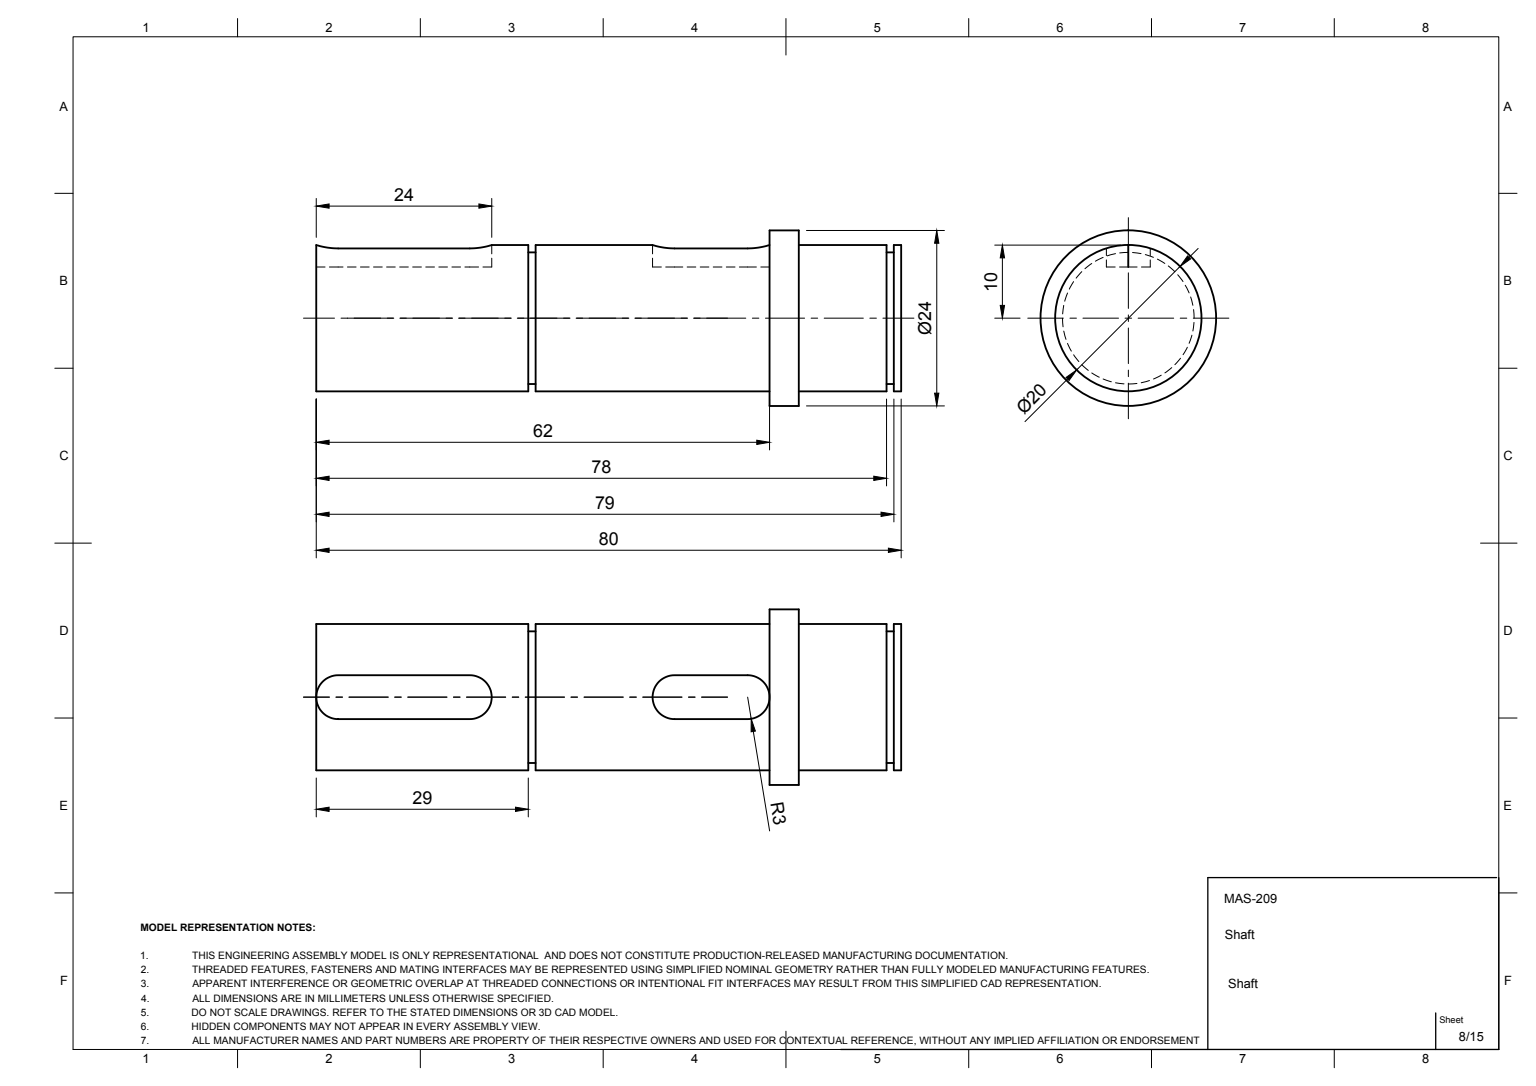
ISO-10303-21;
HEADER;
/* Generated by software containing ST-Developer
 * from STEP Tools, Inc. (www.steptools.com) 
 */

FILE_DESCRIPTION(
/* description */ ('Independent bearing-supported roller-ramp one-way clutch. Six logarit
hmic ramps with plain solid rollers, sprung guided plungers, native Co
il variants, removable shared keepers, rounded parallel key, shaft wit
h complete retaining lips, bronze journal/thrust support and bolted co
vers. Native rotor, roller planar/spin and plunger joints permit manua
l geometric engaged/released inspection. Automatic frictional torque s
witching/contact dynamics are not simulated; no capacity, hardness, fi
t, lubrication, speed, force or life rating. External input driver/cou
pling/anchors outside assembly.'),
/* implementation_level */ '2;1');

FILE_NAME(
/* name */ 'Shaft.step',
/* time_stamp */ '2026-11-08T07:04:38-08:00',
/* author */ (''),
/* organization */ (''),
/* preprocessor_version */ 'ST-DEVELOPER v20.2',
/* originating_system */ 'Autodesk Translation Framework v15.17.0.0',
/* authorisation */ '');

FILE_SCHEMA (('AUTOMOTIVE_DESIGN { 1 0 10303 214 3 1 1 }'));
ENDSEC;

DATA;
#10=MECHANICAL_DESIGN_GEOMETRIC_PRESENTATION_REPRESENTATION('',(#302),#99526);
#270=SHAPE_REPRESENTATION_RELATIONSHIP('SRR','None',#99627,#286);
#286=ADVANCED_BREP_SHAPE_REPRESENTATION('',(#318),#99512);
#302=STYLED_ITEM('',(#99716),#318);
#318=MANIFOLD_SOLID_BREP('Body1',#18272);
#388=FACE_BOUND('',#2557,.T.);
#389=FACE_BOUND('',#2559,.T.);
#390=FACE_BOUND('',#2562,.T.);
#391=FACE_BOUND('',#2564,.T.);
#392=FACE_BOUND('',#2567,.T.);
#393=FACE_BOUND('',#2569,.T.);
#547=PLANE('',#19435);
#548=PLANE('',#19438);
#549=PLANE('',#19439);
#550=PLANE('',#19446);
#551=PLANE('',#19449);
#552=PLANE('',#19450);
#553=PLANE('',#19458);
#554=PLANE('',#19459);
#555=PLANE('',#19463);
#556=PLANE('',#19465);
#557=PLANE('',#19469);
#558=PLANE('',#19471);
#559=PLANE('',#19476);
#560=PLANE('',#19477);
#1489=FACE_OUTER_BOUND('',#2542,.T.);
#1490=FACE_OUTER_BOUND('',#2543,.T.);
#1491=FACE_OUTER_BOUND('',#2544,.T.);
#1492=FACE_OUTER_BOUND('',#2545,.T.);
#1493=FACE_OUTER_BOUND('',#2546,.T.);
#1494=FACE_OUTER_BOUND('',#2547,.T.);
#1495=FACE_OUTER_BOUND('',#2548,.T.);
#1496=FACE_OUTER_BOUND('',#2549,.T.);
#1497=FACE_OUTER_BOUND('',#2550,.T.);
#1498=FACE_OUTER_BOUND('',#2551,.T.);
#1499=FACE_OUTER_BOUND('',#2552,.T.);
#1500=FACE_OUTER_BOUND('',#2553,.T.);
#1501=FACE_OUTER_BOUND('',#2554,.T.);
#1502=FACE_OUTER_BOUND('',#2555,.T.);
#1503=FACE_OUTER_BOUND('',#2556,.T.);
#1504=FACE_OUTER_BOUND('',#2558,.T.);
#1505=FACE_OUTER_BOUND('',#2560,.T.);
#1506=FACE_OUTER_BOUND('',#2561,.T.);
#1507=FACE_OUTER_BOUND('',#2563,.T.);
#1508=FACE_OUTER_BOUND('',#2565,.T.);
#1509=FACE_OUTER_BOUND('',#2566,.T.);
#1510=FACE_OUTER_BOUND('',#2568,.T.);
#1511=FACE_OUTER_BOUND('',#2570,.T.);
#1512=FACE_OUTER_BOUND('',#2571,.T.);
#1513=FACE_OUTER_BOUND('',#2572,.T.);
#1514=FACE_OUTER_BOUND('',#2573,.T.);
#2542=EDGE_LOOP('',(#15718,#15719,#15720,#15721));
#2543=EDGE_LOOP('',(#15722,#15723,#15724,#15725));
#2544=EDGE_LOOP('',(#15726,#15727,#15728,#15729));
#2545=EDGE_LOOP('',(#15730,#15731,#15732,#15733));
#2546=EDGE_LOOP('',(#15734,#15735,#15736,#15737));
#2547=EDGE_LOOP('',(#15738,#15739,#15740,#15741,#15742));
#2548=EDGE_LOOP('',(#15743,#15744,#15745,#15746,#15747,#15748,#15749,#15750,
#15751,#15752));
#2549=EDGE_LOOP('',(#15753,#15754,#15755,#15756));
#2550=EDGE_LOOP('',(#15757,#15758,#15759,#15760));
#2551=EDGE_LOOP('',(#15761,#15762,#15763,#15764,#15765));
#2552=EDGE_LOOP('',(#15766,#15767,#15768,#15769));
#2553=EDGE_LOOP('',(#15770,#15771,#15772,#15773));
#2554=EDGE_LOOP('',(#15774,#15775,#15776,#15777,#15778,#15779,#15780,#15781,
#15782,#15783));
#2555=EDGE_LOOP('',(#15784,#15785,#15786,#15787));
#2556=EDGE_LOOP('',(#15788));
#2557=EDGE_LOOP('',(#15789));
#2558=EDGE_LOOP('',(#15790));
#2559=EDGE_LOOP('',(#15791));
#2560=EDGE_LOOP('',(#15792,#15793,#15794,#15795));
#2561=EDGE_LOOP('',(#15796));
#2562=EDGE_LOOP('',(#15797));
#2563=EDGE_LOOP('',(#15798));
#2564=EDGE_LOOP('',(#15799));
#2565=EDGE_LOOP('',(#15800,#15801,#15802,#15803));
#2566=EDGE_LOOP('',(#15804));
#2567=EDGE_LOOP('',(#15805,#15806));
#2568=EDGE_LOOP('',(#15807));
#2569=EDGE_LOOP('',(#15808));
#2570=EDGE_LOOP('',(#15809,#15810,#15811,#15812));
#2571=EDGE_LOOP('',(#15813,#15814,#15815,#15816));
#2572=EDGE_LOOP('',(#15817,#15818,#15819,#15820));
#2573=EDGE_LOOP('',(#15821));
#2995=CIRCLE('',#19432,3.);
#2996=CIRCLE('',#19434,3.);
#2997=CIRCLE('',#19437,3.);
#2998=CIRCLE('',#19441,10.);
#2999=CIRCLE('',#19442,10.);
#3000=CIRCLE('',#19443,10.);
#3001=CIRCLE('',#19445,3.);
#3002=CIRCLE('',#19448,3.);
#3003=CIRCLE('',#19452,10.);
#3004=CIRCLE('',#19453,10.);
#3005=CIRCLE('',#19454,10.);
#3006=CIRCLE('',#19456,9.);
#3007=CIRCLE('',#19457,9.);
#3008=CIRCLE('',#19461,9.);
#3009=CIRCLE('',#19462,9.);
#3010=CIRCLE('',#19464,10.);
#3011=CIRCLE('',#19466,10.);
#3012=CIRCLE('',#19468,10.);
#3013=CIRCLE('',#19470,12.);
#3014=CIRCLE('',#19472,12.);
#3015=CIRCLE('',#19475,10.);
#4509=B_SPLINE_CURVE_WITH_KNOTS('',3,(#94457,#94458,#94459,#94460,#94461,
#94462,#94463,#94464,#94465,#94466),.UNSPECIFIED.,.F.,.F.,(4,2,2,2,4),(-0.455064911568751,
-0.34131563198115,-0.227566352393549,-0.113783176196775,0.),
 .UNSPECIFIED.);
#4510=B_SPLINE_CURVE_WITH_KNOTS('',3,(#94469,#94470,#94471,#94472,#94473,
#94474,#94475,#94476,#94477,#94478),.UNSPECIFIED.,.F.,.F.,(4,2,2,2,4),(-0.910129823137502,
-0.796346646940727,-0.682563470743952,-0.568814191156351,-0.455064911568751),
 .UNSPECIFIED.);
#4511=B_SPLINE_CURVE_WITH_KNOTS('',3,(#94491,#94492,#94493,#94494,#94495,
#94496,#94497,#94498,#94499,#94500,#94501,#94502,#94503,#94504,#94505,#94506,
#94507,#94508),.UNSPECIFIED.,.F.,.F.,(4,2,2,2,2,2,2,2,4),(0.,0.113783176196775,
0.227566352393549,0.34131563198115,0.455064911568751,0.568814191156351,
0.682563470743952,0.796346646940727,0.910129823137502),.UNSPECIFIED.);
#4512=B_SPLINE_CURVE_WITH_KNOTS('',3,(#94526,#94527,#94528,#94529,#94530,
#94531,#94532,#94533,#94534,#94535,#94536,#94537,#94538,#94539,#94540,#94541,
#94542,#94543),.UNSPECIFIED.,.F.,.F.,(4,2,2,2,2,2,2,2,4),(-0.910129823137503,
-0.796346646940728,-0.682563470743953,-0.568814191156352,-0.455064911568751,
-0.341315631981151,-0.22756635239355,-0.113783176196775,0.),
 .UNSPECIFIED.);
#4513=B_SPLINE_CURVE_WITH_KNOTS('',3,(#94558,#94559,#94560,#94561,#94562,
#94563,#94564,#94565,#94566,#94567),.UNSPECIFIED.,.F.,.F.,(4,2,2,2,4),(0.455064911568751,
0.568814191156352,0.682563470743953,0.796346646940727,0.910129823137502),
 .UNSPECIFIED.);
#4514=B_SPLINE_CURVE_WITH_KNOTS('',3,(#94568,#94569,#94570,#94571,#94572,
#94573,#94574,#94575,#94576,#94577),.UNSPECIFIED.,.F.,.F.,(4,2,2,2,4),(0.,
0.113783176196775,0.22756635239355,0.341315631981151,0.455064911568751),
 .UNSPECIFIED.);
#5366=LINE('',#94452,#6270);
#5367=LINE('',#94456,#6271);
#5368=LINE('',#94480,#6272);
#5369=LINE('',#94482,#6273);
#5370=LINE('',#94485,#6274);
#5371=LINE('',#94487,#6275);
#5372=LINE('',#94488,#6276);
#5373=LINE('',#94511,#6277);
#5374=LINE('',#94513,#6278);
#5375=LINE('',#94514,#6279);
#5376=LINE('',#94521,#6280);
#5377=LINE('',#94545,#6281);
#5378=LINE('',#94548,#6282);
#5379=LINE('',#94551,#6283);
#5380=LINE('',#94553,#6284);
#5381=LINE('',#94554,#6285);
#5382=LINE('',#94580,#6286);
#5383=LINE('',#94582,#6287);
#5384=LINE('',#94583,#6288);
#5385=LINE('',#94589,#6289);
#5386=LINE('',#94596,#6290);
#5387=LINE('',#94604,#6291);
#5388=LINE('',#94615,#6292);
#5389=LINE('',#94623,#6293);
#5390=LINE('',#94626,#6294);
#6270=VECTOR('',#22473,10.);
#6271=VECTOR('',#22476,10.);
#6272=VECTOR('',#22479,10.);
#6273=VECTOR('',#22482,10.);
#6274=VECTOR('',#22485,10.);
#6275=VECTOR('',#22486,10.);
#6276=VECTOR('',#22487,10.);
#6277=VECTOR('',#22492,10.);
#6278=VECTOR('',#22495,10.);
#6279=VECTOR('',#22496,10.);
#6280=VECTOR('',#22505,10.);
#6281=VECTOR('',#22510,10.);
#6282=VECTOR('',#22513,10.);
#6283=VECTOR('',#22516,10.);
#6284=VECTOR('',#22517,10.);
#6285=VECTOR('',#22518,10.);
#6286=VECTOR('',#22523,10.);
#6287=VECTOR('',#22526,10.);
#6288=VECTOR('',#22527,10.);
#6289=VECTOR('',#22534,10.);
#6290=VECTOR('',#22543,9.);
#6291=VECTOR('',#22554,9.);
#6292=VECTOR('',#22569,10.);
#6293=VECTOR('',#22580,12.);
#6294=VECTOR('',#22583,10.);
#7994=VERTEX_POINT('',#94450);
#7995=VERTEX_POINT('',#94451);
#7996=VERTEX_POINT('',#94453);
#7997=VERTEX_POINT('',#94455);
#7998=VERTEX_POINT('',#94468);
#7999=VERTEX_POINT('',#94479);
#8000=VERTEX_POINT('',#94484);
#8001=VERTEX_POINT('',#94486);
#8002=VERTEX_POINT('',#94490);
#8003=VERTEX_POINT('',#94509);
#8004=VERTEX_POINT('',#94517);
#8005=VERTEX_POINT('',#94520);
#8006=VERTEX_POINT('',#94524);
#8007=VERTEX_POINT('',#94525);
#8008=VERTEX_POINT('',#94544);
#8009=VERTEX_POINT('',#94546);
#8010=VERTEX_POINT('',#94550);
#8011=VERTEX_POINT('',#94552);
#8012=VERTEX_POINT('',#94556);
#8013=VERTEX_POINT('',#94557);
#8014=VERTEX_POINT('',#94578);
#8015=VERTEX_POINT('',#94586);
#8016=VERTEX_POINT('',#94588);
#8017=VERTEX_POINT('',#94593);
#8018=VERTEX_POINT('',#94595);
#8019=VERTEX_POINT('',#94601);
#8020=VERTEX_POINT('',#94603);
#8021=VERTEX_POINT('',#94607);
#8022=VERTEX_POINT('',#94610);
#8023=VERTEX_POINT('',#94613);
#8024=VERTEX_POINT('',#94617);
#8025=VERTEX_POINT('',#94620);
#8026=VERTEX_POINT('',#94625);
#10611=EDGE_CURVE('',#7994,#7995,#5366,.T.);
#10612=EDGE_CURVE('',#7996,#7994,#2995,.T.);
#10613=EDGE_CURVE('',#7996,#7997,#5367,.T.);
#10614=EDGE_CURVE('',#7995,#7997,#4509,.T.);
#10615=EDGE_CURVE('',#7998,#7995,#4510,.T.);
#10616=EDGE_CURVE('',#7999,#7998,#5368,.T.);
#10617=EDGE_CURVE('',#7994,#7999,#2996,.T.);
#10618=EDGE_CURVE('',#7994,#7995,#5369,.T.);
#10619=EDGE_CURVE('',#7997,#8000,#5370,.T.);
#10620=EDGE_CURVE('',#7996,#8001,#5371,.T.);
#10621=EDGE_CURVE('',#8001,#8000,#5372,.T.);
#10622=EDGE_CURVE('',#8000,#8002,#4511,.T.);
#10623=EDGE_CURVE('',#8003,#8001,#2997,.T.);
#10624=EDGE_CURVE('',#8003,#8002,#5373,.T.);
#10625=EDGE_CURVE('',#8002,#7998,#5374,.T.);
#10626=EDGE_CURVE('',#8003,#7999,#5375,.T.);
#10627=EDGE_CURVE('',#7995,#8004,#2998,.T.);
#10628=EDGE_CURVE('',#8004,#7995,#2999,.T.);
#10629=EDGE_CURVE('',#8004,#8005,#5376,.T.);
#10630=EDGE_CURVE('',#8005,#8005,#3000,.T.);
#10631=EDGE_CURVE('',#8006,#8007,#4512,.T.);
#10632=EDGE_CURVE('',#8008,#8006,#5377,.T.);
#10633=EDGE_CURVE('',#8009,#8008,#3001,.T.);
#10634=EDGE_CURVE('',#8009,#8007,#5378,.T.);
#10635=EDGE_CURVE('',#8007,#8010,#5379,.T.);
#10636=EDGE_CURVE('',#8009,#8011,#5380,.T.);
#10637=EDGE_CURVE('',#8011,#8010,#5381,.T.);
#10638=EDGE_CURVE('',#8012,#8013,#4513,.T.);
#10639=EDGE_CURVE('',#8010,#8012,#4514,.T.);
#10640=EDGE_CURVE('',#8014,#8011,#3002,.T.);
#10641=EDGE_CURVE('',#8014,#8013,#5382,.T.);
#10642=EDGE_CURVE('',#8013,#8006,#5383,.T.);
#10643=EDGE_CURVE('',#8014,#8008,#5384,.T.);
#10644=EDGE_CURVE('',#8015,#8015,#3003,.T.);
#10645=EDGE_CURVE('',#8015,#8016,#5385,.T.);
#10646=EDGE_CURVE('',#8016,#8012,#3004,.T.);
#10647=EDGE_CURVE('',#8012,#8016,#3005,.T.);
#10648=EDGE_CURVE('',#8017,#8017,#3006,.T.);
#10649=EDGE_CURVE('',#8017,#8018,#5386,.T.);
#10650=EDGE_CURVE('',#8018,#8018,#3007,.T.);
#10651=EDGE_CURVE('',#8019,#8019,#3008,.T.);
#10652=EDGE_CURVE('',#8019,#8020,#5387,.T.);
#10653=EDGE_CURVE('',#8020,#8020,#3009,.T.);
#10654=EDGE_CURVE('',#8021,#8021,#3010,.T.);
#10655=EDGE_CURVE('',#8022,#8022,#3011,.T.);
#10656=EDGE_CURVE('',#8023,#8023,#3012,.T.);
#10657=EDGE_CURVE('',#8023,#8022,#5388,.T.);
#10658=EDGE_CURVE('',#8024,#8024,#3013,.T.);
#10659=EDGE_CURVE('',#8025,#8025,#3014,.T.);
#10660=EDGE_CURVE('',#8024,#8025,#5389,.T.);
#10661=EDGE_CURVE('',#8021,#8026,#5390,.T.);
#10662=EDGE_CURVE('',#8026,#8026,#3015,.T.);
#15718=ORIENTED_EDGE('',*,*,#10611,.F.);
#15719=ORIENTED_EDGE('',*,*,#10612,.F.);
#15720=ORIENTED_EDGE('',*,*,#10613,.T.);
#15721=ORIENTED_EDGE('',*,*,#10614,.F.);
#15722=ORIENTED_EDGE('',*,*,#10615,.F.);
#15723=ORIENTED_EDGE('',*,*,#10616,.F.);
#15724=ORIENTED_EDGE('',*,*,#10617,.F.);
#15725=ORIENTED_EDGE('',*,*,#10618,.T.);
#15726=ORIENTED_EDGE('',*,*,#10619,.F.);
#15727=ORIENTED_EDGE('',*,*,#10613,.F.);
#15728=ORIENTED_EDGE('',*,*,#10620,.T.);
#15729=ORIENTED_EDGE('',*,*,#10621,.T.);
#15730=ORIENTED_EDGE('',*,*,#10622,.F.);
#15731=ORIENTED_EDGE('',*,*,#10621,.F.);
#15732=ORIENTED_EDGE('',*,*,#10623,.F.);
#15733=ORIENTED_EDGE('',*,*,#10624,.T.);
#15734=ORIENTED_EDGE('',*,*,#10625,.F.);
#15735=ORIENTED_EDGE('',*,*,#10624,.F.);
#15736=ORIENTED_EDGE('',*,*,#10626,.T.);
#15737=ORIENTED_EDGE('',*,*,#10616,.T.);
#15738=ORIENTED_EDGE('',*,*,#10612,.T.);
#15739=ORIENTED_EDGE('',*,*,#10617,.T.);
#15740=ORIENTED_EDGE('',*,*,#10626,.F.);
#15741=ORIENTED_EDGE('',*,*,#10623,.T.);
#15742=ORIENTED_EDGE('',*,*,#10620,.F.);
#15743=ORIENTED_EDGE('',*,*,#10627,.F.);
#15744=ORIENTED_EDGE('',*,*,#10614,.T.);
#15745=ORIENTED_EDGE('',*,*,#10619,.T.);
#15746=ORIENTED_EDGE('',*,*,#10622,.T.);
#15747=ORIENTED_EDGE('',*,*,#10625,.T.);
#15748=ORIENTED_EDGE('',*,*,#10615,.T.);
#15749=ORIENTED_EDGE('',*,*,#10628,.F.);
#15750=ORIENTED_EDGE('',*,*,#10629,.T.);
#15751=ORIENTED_EDGE('',*,*,#10630,.T.);
#15752=ORIENTED_EDGE('',*,*,#10629,.F.);
#15753=ORIENTED_EDGE('',*,*,#10631,.F.);
#15754=ORIENTED_EDGE('',*,*,#10632,.F.);
#15755=ORIENTED_EDGE('',*,*,#10633,.F.);
#15756=ORIENTED_EDGE('',*,*,#10634,.T.);
#15757=ORIENTED_EDGE('',*,*,#10635,.F.);
#15758=ORIENTED_EDGE('',*,*,#10634,.F.);
#15759=ORIENTED_EDGE('',*,*,#10636,.T.);
#15760=ORIENTED_EDGE('',*,*,#10637,.T.);
#15761=ORIENTED_EDGE('',*,*,#10638,.F.);
#15762=ORIENTED_EDGE('',*,*,#10639,.F.);
#15763=ORIENTED_EDGE('',*,*,#10637,.F.);
#15764=ORIENTED_EDGE('',*,*,#10640,.F.);
#15765=ORIENTED_EDGE('',*,*,#10641,.T.);
#15766=ORIENTED_EDGE('',*,*,#10642,.F.);
#15767=ORIENTED_EDGE('',*,*,#10641,.F.);
#15768=ORIENTED_EDGE('',*,*,#10643,.T.);
#15769=ORIENTED_EDGE('',*,*,#10632,.T.);
#15770=ORIENTED_EDGE('',*,*,#10633,.T.);
#15771=ORIENTED_EDGE('',*,*,#10643,.F.);
#15772=ORIENTED_EDGE('',*,*,#10640,.T.);
#15773=ORIENTED_EDGE('',*,*,#10636,.F.);
#15774=ORIENTED_EDGE('',*,*,#10644,.T.);
#15775=ORIENTED_EDGE('',*,*,#10645,.T.);
#15776=ORIENTED_EDGE('',*,*,#10646,.T.);
#15777=ORIENTED_EDGE('',*,*,#10638,.T.);
#15778=ORIENTED_EDGE('',*,*,#10642,.T.);
#15779=ORIENTED_EDGE('',*,*,#10631,.T.);
#15780=ORIENTED_EDGE('',*,*,#10635,.T.);
#15781=ORIENTED_EDGE('',*,*,#10639,.T.);
#15782=ORIENTED_EDGE('',*,*,#10647,.T.);
#15783=ORIENTED_EDGE('',*,*,#10645,.F.);
#15784=ORIENTED_EDGE('',*,*,#10648,.T.);
#15785=ORIENTED_EDGE('',*,*,#10649,.T.);
#15786=ORIENTED_EDGE('',*,*,#10650,.F.);
#15787=ORIENTED_EDGE('',*,*,#10649,.F.);
#15788=ORIENTED_EDGE('',*,*,#10644,.F.);
#15789=ORIENTED_EDGE('',*,*,#10648,.F.);
#15790=ORIENTED_EDGE('',*,*,#10630,.F.);
#15791=ORIENTED_EDGE('',*,*,#10650,.T.);
#15792=ORIENTED_EDGE('',*,*,#10651,.T.);
#15793=ORIENTED_EDGE('',*,*,#10652,.T.);
#15794=ORIENTED_EDGE('',*,*,#10653,.F.);
#15795=ORIENTED_EDGE('',*,*,#10652,.F.);
#15796=ORIENTED_EDGE('',*,*,#10654,.F.);
#15797=ORIENTED_EDGE('',*,*,#10651,.F.);
#15798=ORIENTED_EDGE('',*,*,#10655,.F.);
#15799=ORIENTED_EDGE('',*,*,#10653,.T.);
#15800=ORIENTED_EDGE('',*,*,#10656,.T.);
#15801=ORIENTED_EDGE('',*,*,#10657,.T.);
#15802=ORIENTED_EDGE('',*,*,#10655,.T.);
#15803=ORIENTED_EDGE('',*,*,#10657,.F.);
#15804=ORIENTED_EDGE('',*,*,#10658,.T.);
#15805=ORIENTED_EDGE('',*,*,#10647,.F.);
#15806=ORIENTED_EDGE('',*,*,#10646,.F.);
#15807=ORIENTED_EDGE('',*,*,#10659,.F.);
#15808=ORIENTED_EDGE('',*,*,#10656,.F.);
#15809=ORIENTED_EDGE('',*,*,#10658,.F.);
#15810=ORIENTED_EDGE('',*,*,#10660,.T.);
#15811=ORIENTED_EDGE('',*,*,#10659,.T.);
#15812=ORIENTED_EDGE('',*,*,#10660,.F.);
#15813=ORIENTED_EDGE('',*,*,#10654,.T.);
#15814=ORIENTED_EDGE('',*,*,#10661,.T.);
#15815=ORIENTED_EDGE('',*,*,#10662,.T.);
#15816=ORIENTED_EDGE('',*,*,#10661,.F.);
#15817=ORIENTED_EDGE('',*,*,#10627,.T.);
#15818=ORIENTED_EDGE('',*,*,#10628,.T.);
#15819=ORIENTED_EDGE('',*,*,#10618,.F.);
#15820=ORIENTED_EDGE('',*,*,#10611,.T.);
#15821=ORIENTED_EDGE('',*,*,#10662,.F.);
#17171=CYLINDRICAL_SURFACE('',#19431,3.);
#17172=CYLINDRICAL_SURFACE('',#19433,3.);
#17173=CYLINDRICAL_SURFACE('',#19436,3.);
#17174=CYLINDRICAL_SURFACE('',#19440,10.);
#17175=CYLINDRICAL_SURFACE('',#19444,3.);
#17176=CYLINDRICAL_SURFACE('',#19447,3.);
#17177=CYLINDRICAL_SURFACE('',#19451,10.);
#17178=CYLINDRICAL_SURFACE('',#19455,9.);
#17179=CYLINDRICAL_SURFACE('',#19460,9.);
#17180=CYLINDRICAL_SURFACE('',#19467,10.);
#17181=CYLINDRICAL_SURFACE('',#19473,12.);
#17182=CYLINDRICAL_SURFACE('',#19474,10.);
#18087=ADVANCED_FACE('',(#1489),#17171,.F.);
#18088=ADVANCED_FACE('',(#1490),#17172,.F.);
#18089=ADVANCED_FACE('',(#1491),#547,.F.);
#18090=ADVANCED_FACE('',(#1492),#17173,.F.);
#18091=ADVANCED_FACE('',(#1493),#548,.F.);
#18092=ADVANCED_FACE('',(#1494),#549,.T.);
#18093=ADVANCED_FACE('',(#1495),#17174,.T.);
#18094=ADVANCED_FACE('',(#1496),#17175,.F.);
#18095=ADVANCED_FACE('',(#1497),#550,.F.);
#18096=ADVANCED_FACE('',(#1498),#17176,.F.);
#18097=ADVANCED_FACE('',(#1499),#551,.F.);
#18098=ADVANCED_FACE('',(#1500),#552,.T.);
#18099=ADVANCED_FACE('',(#1501),#17177,.T.);
#18100=ADVANCED_FACE('',(#1502),#17178,.T.);
#18101=ADVANCED_FACE('',(#1503,#388),#553,.F.);
#18102=ADVANCED_FACE('',(#1504,#389),#554,.F.);
#18103=ADVANCED_FACE('',(#1505),#17179,.T.);
#18104=ADVANCED_FACE('',(#1506,#390),#555,.F.);
#18105=ADVANCED_FACE('',(#1507,#391),#556,.F.);
#18106=ADVANCED_FACE('',(#1508),#17180,.T.);
#18107=ADVANCED_FACE('',(#1509,#392),#557,.T.);
#18108=ADVANCED_FACE('',(#1510,#393),#558,.F.);
#18109=ADVANCED_FACE('',(#1511),#17181,.T.);
#18110=ADVANCED_FACE('',(#1512),#17182,.T.);
#18111=ADVANCED_FACE('',(#1513),#559,.T.);
#18112=ADVANCED_FACE('',(#1514),#560,.F.);
#18272=CLOSED_SHELL('',(#18087,#18088,#18089,#18090,#18091,#18092,#18093,
#18094,#18095,#18096,#18097,#18098,#18099,#18100,#18101,#18102,#18103,#18104,
#18105,#18106,#18107,#18108,#18109,#18110,#18111,#18112));
#19430=AXIS2_PLACEMENT_3D('',#94448,#22469,#22470);
#19431=AXIS2_PLACEMENT_3D('',#94449,#22471,#22472);
#19432=AXIS2_PLACEMENT_3D('',#94454,#22474,#22475);
#19433=AXIS2_PLACEMENT_3D('',#94467,#22477,#22478);
#19434=AXIS2_PLACEMENT_3D('',#94481,#22480,#22481);
#19435=AXIS2_PLACEMENT_3D('',#94483,#22483,#22484);
#19436=AXIS2_PLACEMENT_3D('',#94489,#22488,#22489);
#19437=AXIS2_PLACEMENT_3D('',#94510,#22490,#22491);
#19438=AXIS2_PLACEMENT_3D('',#94512,#22493,#22494);
#19439=AXIS2_PLACEMENT_3D('',#94515,#22497,#22498);
#19440=AXIS2_PLACEMENT_3D('',#94516,#22499,#22500);
#19441=AXIS2_PLACEMENT_3D('',#94518,#22501,#22502);
#19442=AXIS2_PLACEMENT_3D('',#94519,#22503,#22504);
#19443=AXIS2_PLACEMENT_3D('',#94522,#22506,#22507);
#19444=AXIS2_PLACEMENT_3D('',#94523,#22508,#22509);
#19445=AXIS2_PLACEMENT_3D('',#94547,#22511,#22512);
#19446=AXIS2_PLACEMENT_3D('',#94549,#22514,#22515);
#19447=AXIS2_PLACEMENT_3D('',#94555,#22519,#22520);
#19448=AXIS2_PLACEMENT_3D('',#94579,#22521,#22522);
#19449=AXIS2_PLACEMENT_3D('',#94581,#22524,#22525);
#19450=AXIS2_PLACEMENT_3D('',#94584,#22528,#22529);
#19451=AXIS2_PLACEMENT_3D('',#94585,#22530,#22531);
#19452=AXIS2_PLACEMENT_3D('',#94587,#22532,#22533);
#19453=AXIS2_PLACEMENT_3D('',#94590,#22535,#22536);
#19454=AXIS2_PLACEMENT_3D('',#94591,#22537,#22538);
#19455=AXIS2_PLACEMENT_3D('',#94592,#22539,#22540);
#19456=AXIS2_PLACEMENT_3D('',#94594,#22541,#22542);
#19457=AXIS2_PLACEMENT_3D('',#94597,#22544,#22545);
#19458=AXIS2_PLACEMENT_3D('',#94598,#22546,#22547);
#19459=AXIS2_PLACEMENT_3D('',#94599,#22548,#22549);
#19460=AXIS2_PLACEMENT_3D('',#94600,#22550,#22551);
#19461=AXIS2_PLACEMENT_3D('',#94602,#22552,#22553);
#19462=AXIS2_PLACEMENT_3D('',#94605,#22555,#22556);
#19463=AXIS2_PLACEMENT_3D('',#94606,#22557,#22558);
#19464=AXIS2_PLACEMENT_3D('',#94608,#22559,#22560);
#19465=AXIS2_PLACEMENT_3D('',#94609,#22561,#22562);
#19466=AXIS2_PLACEMENT_3D('',#94611,#22563,#22564);
#19467=AXIS2_PLACEMENT_3D('',#94612,#22565,#22566);
#19468=AXIS2_PLACEMENT_3D('',#94614,#22567,#22568);
#19469=AXIS2_PLACEMENT_3D('',#94616,#22570,#22571);
#19470=AXIS2_PLACEMENT_3D('',#94618,#22572,#22573);
#19471=AXIS2_PLACEMENT_3D('',#94619,#22574,#22575);
#19472=AXIS2_PLACEMENT_3D('',#94621,#22576,#22577);
#19473=AXIS2_PLACEMENT_3D('',#94622,#22578,#22579);
#19474=AXIS2_PLACEMENT_3D('',#94624,#22581,#22582);
#19475=AXIS2_PLACEMENT_3D('',#94627,#22584,#22585);
#19476=AXIS2_PLACEMENT_3D('',#94628,#22586,#22587);
#19477=AXIS2_PLACEMENT_3D('',#94629,#22588,#22589);
#22469=DIRECTION('axis',(0.,0.,1.));
#22470=DIRECTION('refdir',(1.,0.,0.));
#22471=DIRECTION('center_axis',(1.,0.,0.));
#22472=DIRECTION('ref_axis',(0.,1.,-2.96059473233375E-15));
#22473=DIRECTION('',(1.,0.,0.));
#22474=DIRECTION('center_axis',(1.,0.,0.));
#22475=DIRECTION('ref_axis',(0.,1.,-2.96059473233375E-15));
#22476=DIRECTION('',(1.,0.,0.));
#22477=DIRECTION('center_axis',(1.,0.,0.));
#22478=DIRECTION('ref_axis',(0.,1.,-2.96059473233375E-15));
#22479=DIRECTION('',(1.,0.,0.));
#22480=DIRECTION('center_axis',(1.,0.,0.));
#22481=DIRECTION('ref_axis',(0.,1.,-2.96059473233375E-15));
#22482=DIRECTION('',(1.,0.,0.));
#22483=DIRECTION('center_axis',(0.,1.,0.));
#22484=DIRECTION('ref_axis',(0.,0.,1.));
#22485=DIRECTION('',(0.,0.,-1.));
#22486=DIRECTION('',(0.,0.,-1.));
#22487=DIRECTION('',(1.,0.,0.));
#22488=DIRECTION('center_axis',(1.,0.,0.));
#22489=DIRECTION('ref_axis',(0.,-1.,-2.96059473233375E-15));
#22490=DIRECTION('center_axis',(1.,0.,0.));
#22491=DIRECTION('ref_axis',(0.,-1.,-2.96059473233375E-15));
#22492=DIRECTION('',(1.,0.,0.));
#22493=DIRECTION('center_axis',(0.,-1.,0.));
#22494=DIRECTION('ref_axis',(0.,0.,-1.));
#22495=DIRECTION('',(0.,0.,1.));
#22496=DIRECTION('',(0.,0.,1.));
#22497=DIRECTION('center_axis',(1.,0.,0.));
#22498=DIRECTION('ref_axis',(0.,0.,-1.));
#22499=DIRECTION('center_axis',(0.,0.,1.));
#22500=DIRECTION('ref_axis',(1.,0.,0.));
#22501=DIRECTION('center_axis',(0.,0.,1.));
#22502=DIRECTION('ref_axis',(1.,0.,0.));
#22503=DIRECTION('center_axis',(0.,0.,1.));
#22504=DIRECTION('ref_axis',(1.,0.,0.));
#22505=DIRECTION('',(0.,0.,-1.));
#22506=DIRECTION('center_axis',(0.,0.,1.));
#22507=DIRECTION('ref_axis',(1.,0.,0.));
#22508=DIRECTION('center_axis',(1.,0.,0.));
#22509=DIRECTION('ref_axis',(0.,1.,0.));
#22510=DIRECTION('',(1.,0.,0.));
#22511=DIRECTION('center_axis',(1.,0.,0.));
#22512=DIRECTION('ref_axis',(0.,1.,0.));
#22513=DIRECTION('',(1.,0.,0.));
#22514=DIRECTION('center_axis',(0.,1.,0.));
#22515=DIRECTION('ref_axis',(0.,0.,1.));
#22516=DIRECTION('',(0.,0.,-1.));
#22517=DIRECTION('',(0.,0.,-1.));
#22518=DIRECTION('',(1.,0.,0.));
#22519=DIRECTION('center_axis',(1.,0.,0.));
#22520=DIRECTION('ref_axis',(0.,-1.,0.));
#22521=DIRECTION('center_axis',(1.,0.,0.));
#22522=DIRECTION('ref_axis',(0.,-1.,0.));
#22523=DIRECTION('',(1.,0.,0.));
#22524=DIRECTION('center_axis',(0.,-1.,0.));
#22525=DIRECTION('ref_axis',(0.,0.,-1.));
#22526=DIRECTION('',(0.,0.,1.));
#22527=DIRECTION('',(0.,0.,1.));
#22528=DIRECTION('center_axis',(1.,0.,0.));
#22529=DIRECTION('ref_axis',(0.,0.,-1.));
#22530=DIRECTION('center_axis',(0.,0.,1.));
#22531=DIRECTION('ref_axis',(1.,0.,0.));
#22532=DIRECTION('center_axis',(0.,0.,-1.));
#22533=DIRECTION('ref_axis',(1.,0.,0.));
#22534=DIRECTION('',(0.,0.,-1.));
#22535=DIRECTION('center_axis',(0.,0.,1.));
#22536=DIRECTION('ref_axis',(1.,0.,0.));
#22537=DIRECTION('center_axis',(0.,0.,1.));
#22538=DIRECTION('ref_axis',(1.,0.,0.));
#22539=DIRECTION('center_axis',(0.,0.,1.));
#22540=DIRECTION('ref_axis',(1.,0.,0.));
#22541=DIRECTION('center_axis',(0.,0.,1.));
#22542=DIRECTION('ref_axis',(1.,0.,0.));
#22543=DIRECTION('',(0.,0.,1.));
#22544=DIRECTION('center_axis',(0.,0.,1.));
#22545=DIRECTION('ref_axis',(1.,0.,0.));
#22546=DIRECTION('center_axis',(0.,0.,-1.));
#22547=DIRECTION('ref_axis',(-1.,0.,0.));
#22548=DIRECTION('center_axis',(0.,0.,1.));
#22549=DIRECTION('ref_axis',(1.,0.,0.));
#22550=DIRECTION('center_axis',(0.,0.,1.));
#22551=DIRECTION('ref_axis',(1.,0.,0.));
#22552=DIRECTION('center_axis',(0.,0.,1.));
#22553=DIRECTION('ref_axis',(1.,0.,0.));
#22554=DIRECTION('',(0.,0.,1.));
#22555=DIRECTION('center_axis',(0.,0.,1.));
#22556=DIRECTION('ref_axis',(1.,0.,0.));
#22557=DIRECTION('center_axis',(0.,0.,-1.));
#22558=DIRECTION('ref_axis',(-1.,0.,0.));
#22559=DIRECTION('center_axis',(0.,0.,-1.));
#22560=DIRECTION('ref_axis',(1.,0.,0.));
#22561=DIRECTION('center_axis',(0.,0.,1.));
#22562=DIRECTION('ref_axis',(1.,0.,0.));
#22563=DIRECTION('center_axis',(0.,0.,1.));
#22564=DIRECTION('ref_axis',(1.,0.,0.));
#22565=DIRECTION('center_axis',(0.,0.,1.));
#22566=DIRECTION('ref_axis',(1.,0.,0.));
#22567=DIRECTION('center_axis',(0.,0.,-1.));
#22568=DIRECTION('ref_axis',(1.,0.,0.));
#22569=DIRECTION('',(0.,0.,-1.));
#22570=DIRECTION('center_axis',(0.,0.,1.));
#22571=DIRECTION('ref_axis',(1.,0.,0.));
#22572=DIRECTION('center_axis',(0.,0.,1.));
#22573=DIRECTION('ref_axis',(1.,0.,0.));
#22574=DIRECTION('center_axis',(0.,0.,1.));
#22575=DIRECTION('ref_axis',(1.,0.,0.));
#22576=DIRECTION('center_axis',(0.,0.,1.));
#22577=DIRECTION('ref_axis',(1.,0.,0.));
#22578=DIRECTION('center_axis',(0.,0.,1.));
#22579=DIRECTION('ref_axis',(1.,0.,0.));
#22580=DIRECTION('',(0.,0.,-1.));
#22581=DIRECTION('center_axis',(0.,0.,1.));
#22582=DIRECTION('ref_axis',(1.,0.,0.));
#22583=DIRECTION('',(0.,0.,-1.));
#22584=DIRECTION('center_axis',(0.,0.,1.));
#22585=DIRECTION('ref_axis',(1.,0.,0.));
#22586=DIRECTION('center_axis',(0.,0.,1.));
#22587=DIRECTION('ref_axis',(1.,0.,0.));
#22588=DIRECTION('center_axis',(0.,0.,1.));
#22589=DIRECTION('ref_axis',(1.,0.,0.));
#94448=CARTESIAN_POINT('',(0.,0.,0.));
#94449=CARTESIAN_POINT('Origin',(7.,0.,61.));
#94450=CARTESIAN_POINT('',(7.,0.,64.));
#94451=CARTESIAN_POINT('',(10.,0.,64.));
#94452=CARTESIAN_POINT('',(7.,0.,64.));
#94453=CARTESIAN_POINT('',(7.,3.,61.));
#94454=CARTESIAN_POINT('Origin',(7.,0.,61.));
#94455=CARTESIAN_POINT('',(9.53939201416946,3.,61.));
#94456=CARTESIAN_POINT('',(7.,3.,61.));
#94457=CARTESIAN_POINT('Ctrl Pts',(10.,2.77555756156289E-16,64.));
#94458=CARTESIAN_POINT('Ctrl Pts',(10.,0.379164265292003,64.));
#94459=CARTESIAN_POINT('Ctrl Pts',(9.97630133387832,0.782037717481879,63.9237482465107));
#94460=CARTESIAN_POINT('Ctrl Pts',(9.8907119499008,1.52052241900623,63.616848907033));
#94461=CARTESIAN_POINT('Ctrl Pts',(9.82993562614982,1.85631434471708,63.3863263424022));
#94462=CARTESIAN_POINT('Ctrl Pts',(9.71486751729016,2.38640531261462,62.8562353745047));
#94463=CARTESIAN_POINT('Ctrl Pts',(9.65284956103208,2.61686672615765,62.5204755377162));
#94464=CARTESIAN_POINT('Ctrl Pts',(9.56437939057488,2.92372091609921,61.7821074854282));
#94465=CARTESIAN_POINT('Ctrl Pts',(9.53939201416946,3.,61.3792772539893));
#94466=CARTESIAN_POINT('Ctrl Pts',(9.53939201416946,3.,61.));
#94467=CARTESIAN_POINT('Origin',(7.,0.,61.));
#94468=CARTESIAN_POINT('',(9.53939201416946,-3.,61.));
#94469=CARTESIAN_POINT('Ctrl Pts',(9.53939201416946,-3.,61.));
#94470=CARTESIAN_POINT('Ctrl Pts',(9.53939201416946,-3.,61.3792772539893));
#94471=CARTESIAN_POINT('Ctrl Pts',(9.56437939057487,-2.92372091609922,61.7821074854282));
#94472=CARTESIAN_POINT('Ctrl Pts',(9.65284956103208,-2.61686672615766,62.5204755377161));
#94473=CARTESIAN_POINT('Ctrl Pts',(9.71486751729016,-2.38640531261463,62.8562353745047));
#94474=CARTESIAN_POINT('Ctrl Pts',(9.82993562614982,-1.85631434471708,63.3863263424022));
#94475=CARTESIAN_POINT('Ctrl Pts',(9.8907119499008,-1.52052241900622,63.616848907033));
#94476=CARTESIAN_POINT('Ctrl Pts',(9.97630133387832,-0.782037717481873,
63.9237482465107));
#94477=CARTESIAN_POINT('Ctrl Pts',(10.,-0.379164265292002,64.));
#94478=CARTESIAN_POINT('Ctrl Pts',(10.,-5.55111512312578E-16,64.));
#94479=CARTESIAN_POINT('',(7.,-3.,61.));
#94480=CARTESIAN_POINT('',(7.,-3.,61.));
#94481=CARTESIAN_POINT('Origin',(7.,0.,61.));
#94482=CARTESIAN_POINT('',(7.,0.,64.));
#94483=CARTESIAN_POINT('Origin',(7.,3.,43.));
#94484=CARTESIAN_POINT('',(9.53939201416946,3.,43.));
#94485=CARTESIAN_POINT('',(9.53939201416946,3.,-16.));
#94486=CARTESIAN_POINT('',(7.,3.,43.));
#94487=CARTESIAN_POINT('',(7.,3.,61.));
#94488=CARTESIAN_POINT('',(7.,3.,43.));
#94489=CARTESIAN_POINT('Origin',(7.,-2.77555756156289E-16,43.));
#94490=CARTESIAN_POINT('',(9.53939201416946,-3.,43.));
#94491=CARTESIAN_POINT('Ctrl Pts',(9.53939201416946,3.,43.));
#94492=CARTESIAN_POINT('Ctrl Pts',(9.53939201416946,3.,42.6207227460108));
#94493=CARTESIAN_POINT('Ctrl Pts',(9.56437939057488,2.92372091609922,42.2178925145718));
#94494=CARTESIAN_POINT('Ctrl Pts',(9.65284956103208,2.61686672615766,41.4795244622839));
#94495=CARTESIAN_POINT('Ctrl Pts',(9.71486751729016,2.38640531261462,41.1437646254954));
#94496=CARTESIAN_POINT('Ctrl Pts',(9.82993562614982,1.85631434471708,40.6136736575978));
#94497=CARTESIAN_POINT('Ctrl Pts',(9.8907119499008,1.52052241900622,40.383151092967));
#94498=CARTESIAN_POINT('Ctrl Pts',(9.97630133387832,0.78203771748188,40.0762517534893));
#94499=CARTESIAN_POINT('Ctrl Pts',(10.,0.379164265292002,40.));
#94500=CARTESIAN_POINT('Ctrl Pts',(10.,-0.379164265292002,40.));
#94501=CARTESIAN_POINT('Ctrl Pts',(9.97630133387832,-0.782037717481879,
40.0762517534893));
#94502=CARTESIAN_POINT('Ctrl Pts',(9.8907119499008,-1.52052241900622,40.383151092967));
#94503=CARTESIAN_POINT('Ctrl Pts',(9.82993562614982,-1.85631434471708,40.6136736575978));
#94504=CARTESIAN_POINT('Ctrl Pts',(9.71486751729016,-2.38640531261463,41.1437646254954));
#94505=CARTESIAN_POINT('Ctrl Pts',(9.65284956103208,-2.61686672615766,41.4795244622839));
#94506=CARTESIAN_POINT('Ctrl Pts',(9.56437939057488,-2.92372091609922,42.2178925145718));
#94507=CARTESIAN_POINT('Ctrl Pts',(9.53939201416946,-3.,42.6207227460108));
#94508=CARTESIAN_POINT('Ctrl Pts',(9.53939201416946,-3.,43.));
#94509=CARTESIAN_POINT('',(7.,-3.,43.));
#94510=CARTESIAN_POINT('Origin',(7.,-2.77555756156289E-16,43.));
#94511=CARTESIAN_POINT('',(7.,-3.,43.));
#94512=CARTESIAN_POINT('Origin',(7.,-3.,61.));
#94513=CARTESIAN_POINT('',(9.53939201416946,-3.,-16.));
#94514=CARTESIAN_POINT('',(7.,-3.,43.));
#94515=CARTESIAN_POINT('Origin',(7.,0.,52.));
#94516=CARTESIAN_POINT('Origin',(0.,0.,-16.));
#94517=CARTESIAN_POINT('',(-10.,-1.22464679914735E-15,64.));
#94518=CARTESIAN_POINT('Origin',(0.,0.,64.));
#94519=CARTESIAN_POINT('Origin',(0.,0.,64.));
#94520=CARTESIAN_POINT('',(-10.,-1.22464679914735E-15,35.));
#94521=CARTESIAN_POINT('',(-10.,-1.22464679914735E-15,-16.));
#94522=CARTESIAN_POINT('Origin',(0.,0.,35.));
#94523=CARTESIAN_POINT('Origin',(7.,0.,15.));
#94524=CARTESIAN_POINT('',(9.53939201416946,-3.,15.));
#94525=CARTESIAN_POINT('',(9.53939201416946,3.,15.));
#94526=CARTESIAN_POINT('Ctrl Pts',(9.53939201416946,-3.,15.));
#94527=CARTESIAN_POINT('Ctrl Pts',(9.53939201416946,-3.,15.3792772539892));
#94528=CARTESIAN_POINT('Ctrl Pts',(9.56437939057488,-2.92372091609922,15.7821074854282));
#94529=CARTESIAN_POINT('Ctrl Pts',(9.65284956103208,-2.61686672615765,16.5204755377161));
#94530=CARTESIAN_POINT('Ctrl Pts',(9.71486751729016,-2.38640531261463,16.8562353745047));
#94531=CARTESIAN_POINT('Ctrl Pts',(9.82993562614982,-1.85631434471708,17.3863263424022));
#94532=CARTESIAN_POINT('Ctrl Pts',(9.8907119499008,-1.52052241900622,17.616848907033));
#94533=CARTESIAN_POINT('Ctrl Pts',(9.97630133387832,-0.782037717481878,
17.9237482465107));
#94534=CARTESIAN_POINT('Ctrl Pts',(10.,-0.379164265292003,18.));
#94535=CARTESIAN_POINT('Ctrl Pts',(10.,0.379164265292001,18.));
#94536=CARTESIAN_POINT('Ctrl Pts',(9.97630133387832,0.782037717481875,17.9237482465107));
#94537=CARTESIAN_POINT('Ctrl Pts',(9.8907119499008,1.52052241900622,17.616848907033));
#94538=CARTESIAN_POINT('Ctrl Pts',(9.82993562614982,1.85631434471708,17.3863263424022));
#94539=CARTESIAN_POINT('Ctrl Pts',(9.71486751729016,2.38640531261462,16.8562353745047));
#94540=CARTESIAN_POINT('Ctrl Pts',(9.65284956103208,2.61686672615765,16.5204755377161));
#94541=CARTESIAN_POINT('Ctrl Pts',(9.56437939057488,2.92372091609922,15.7821074854282));
#94542=CARTESIAN_POINT('Ctrl Pts',(9.53939201416946,3.,15.3792772539892));
#94543=CARTESIAN_POINT('Ctrl Pts',(9.53939201416946,3.,15.));
#94544=CARTESIAN_POINT('',(7.,-3.,15.));
#94545=CARTESIAN_POINT('',(7.,-3.,15.));
#94546=CARTESIAN_POINT('',(7.,3.,15.));
#94547=CARTESIAN_POINT('Origin',(7.,0.,15.));
#94548=CARTESIAN_POINT('',(7.,3.,15.));
#94549=CARTESIAN_POINT('Origin',(7.,3.,5.));
#94550=CARTESIAN_POINT('',(9.53939201416946,3.,5.));
#94551=CARTESIAN_POINT('',(9.53939201416946,3.,-16.));
#94552=CARTESIAN_POINT('',(7.,3.,5.));
#94553=CARTESIAN_POINT('',(7.,3.,15.));
#94554=CARTESIAN_POINT('',(7.,3.,5.));
#94555=CARTESIAN_POINT('Origin',(7.,0.,5.));
#94556=CARTESIAN_POINT('',(10.,0.,2.));
#94557=CARTESIAN_POINT('',(9.53939201416946,-3.,5.));
#94558=CARTESIAN_POINT('Ctrl Pts',(10.,-2.77555756156289E-16,2.));
#94559=CARTESIAN_POINT('Ctrl Pts',(10.,-0.379164265292002,2.));
#94560=CARTESIAN_POINT('Ctrl Pts',(9.97630133387832,-0.782037717481877,
2.07625175348933));
#94561=CARTESIAN_POINT('Ctrl Pts',(9.8907119499008,-1.52052241900622,2.38315109296703));
#94562=CARTESIAN_POINT('Ctrl Pts',(9.82993562614982,-1.85631434471708,2.61367365759779));
#94563=CARTESIAN_POINT('Ctrl Pts',(9.71486751729016,-2.38640531261463,3.14376462549534));
#94564=CARTESIAN_POINT('Ctrl Pts',(9.65284956103208,-2.61686672615765,3.47952446228385));
#94565=CARTESIAN_POINT('Ctrl Pts',(9.56437939057488,-2.92372091609922,4.21789251457176));
#94566=CARTESIAN_POINT('Ctrl Pts',(9.53939201416946,-3.,4.62072274601075));
#94567=CARTESIAN_POINT('Ctrl Pts',(9.53939201416946,-3.,5.));
#94568=CARTESIAN_POINT('Ctrl Pts',(9.53939201416946,3.,5.));
#94569=CARTESIAN_POINT('Ctrl Pts',(9.53939201416946,3.,4.62072274601075));
#94570=CARTESIAN_POINT('Ctrl Pts',(9.56437939057488,2.92372091609922,4.21789251457176));
#94571=CARTESIAN_POINT('Ctrl Pts',(9.65284956103208,2.61686672615765,3.47952446228385));
#94572=CARTESIAN_POINT('Ctrl Pts',(9.71486751729016,2.38640531261463,3.14376462549534));
#94573=CARTESIAN_POINT('Ctrl Pts',(9.82993562614982,1.85631434471708,2.61367365759779));
#94574=CARTESIAN_POINT('Ctrl Pts',(9.8907119499008,1.52052241900622,2.38315109296703));
#94575=CARTESIAN_POINT('Ctrl Pts',(9.97630133387832,0.782037717481877,2.07625175348933));
#94576=CARTESIAN_POINT('Ctrl Pts',(10.,0.379164265292002,2.));
#94577=CARTESIAN_POINT('Ctrl Pts',(10.,-4.85722573273506E-16,2.));
#94578=CARTESIAN_POINT('',(7.,-3.,5.));
#94579=CARTESIAN_POINT('Origin',(7.,0.,5.));
#94580=CARTESIAN_POINT('',(7.,-3.,5.));
#94581=CARTESIAN_POINT('Origin',(7.,-3.,15.));
#94582=CARTESIAN_POINT('',(9.53939201416946,-3.,-16.));
#94583=CARTESIAN_POINT('',(7.,-3.,5.));
#94584=CARTESIAN_POINT('Origin',(7.,0.,10.));
#94585=CARTESIAN_POINT('Origin',(0.,0.,-16.));
#94586=CARTESIAN_POINT('',(-10.,1.22464679914735E-15,34.));
#94587=CARTESIAN_POINT('Origin',(0.,0.,34.));
#94588=CARTESIAN_POINT('',(-10.,-1.22464679914735E-15,2.));
#94589=CARTESIAN_POINT('',(-10.,-1.22464679914735E-15,-16.));
#94590=CARTESIAN_POINT('Origin',(0.,0.,2.));
#94591=CARTESIAN_POINT('Origin',(0.,0.,2.));
#94592=CARTESIAN_POINT('Origin',(0.,0.,34.5));
#94593=CARTESIAN_POINT('',(-9.,-1.10218211923262E-15,34.));
#94594=CARTESIAN_POINT('Origin',(0.,0.,34.));
#94595=CARTESIAN_POINT('',(-9.,-1.10218211923262E-15,35.));
#94596=CARTESIAN_POINT('',(-9.,-1.10218211923262E-15,34.5));
#94597=CARTESIAN_POINT('Origin',(0.,0.,35.));
#94598=CARTESIAN_POINT('Origin',(13.,0.,34.));
#94599=CARTESIAN_POINT('Origin',(9.,0.,35.));
#94600=CARTESIAN_POINT('Origin',(0.,0.,-14.5));
#94601=CARTESIAN_POINT('',(-9.,-1.10218211923262E-15,-15.));
#94602=CARTESIAN_POINT('Origin',(0.,0.,-15.));
#94603=CARTESIAN_POINT('',(-9.,-1.10218211923262E-15,-14.));
#94604=CARTESIAN_POINT('',(-9.,-1.10218211923262E-15,-14.5));
#94605=CARTESIAN_POINT('Origin',(0.,0.,-14.));
#94606=CARTESIAN_POINT('Origin',(13.,0.,-15.));
#94607=CARTESIAN_POINT('',(-10.,1.22464679914735E-15,-15.));
#94608=CARTESIAN_POINT('Origin',(0.,0.,-15.));
#94609=CARTESIAN_POINT('Origin',(9.,0.,-14.));
#94610=CARTESIAN_POINT('',(-10.,-1.22464679914735E-15,-14.));
#94611=CARTESIAN_POINT('Origin',(0.,0.,-14.));
#94612=CARTESIAN_POINT('Origin',(0.,0.,-16.));
#94613=CARTESIAN_POINT('',(-10.,1.22464679914735E-15,-2.));
#94614=CARTESIAN_POINT('Origin',(0.,0.,-2.));
#94615=CARTESIAN_POINT('',(-10.,-1.22464679914735E-15,-16.));
#94616=CARTESIAN_POINT('Origin',(0.,0.,2.));
#94617=CARTESIAN_POINT('',(-12.,-1.46957615897682E-15,2.));
#94618=CARTESIAN_POINT('Origin',(0.,0.,2.));
#94619=CARTESIAN_POINT('Origin',(0.,0.,-2.));
#94620=CARTESIAN_POINT('',(-12.,-1.46957615897682E-15,-2.));
#94621=CARTESIAN_POINT('Origin',(0.,0.,-2.));
#94622=CARTESIAN_POINT('Origin',(0.,0.,-2.));
#94623=CARTESIAN_POINT('',(-12.,-1.46957615897682E-15,-2.));
#94624=CARTESIAN_POINT('Origin',(0.,0.,-16.));
#94625=CARTESIAN_POINT('',(-10.,-1.22464679914735E-15,-16.));
#94626=CARTESIAN_POINT('',(-10.,-1.22464679914735E-15,-16.));
#94627=CARTESIAN_POINT('Origin',(0.,0.,-16.));
#94628=CARTESIAN_POINT('Origin',(0.,0.,64.));
#94629=CARTESIAN_POINT('Origin',(0.,0.,-16.));
#99494=UNCERTAINTY_MEASURE_WITH_UNIT(LENGTH_MEASURE(0.01),#99527,
'DISTANCE_ACCURACY_VALUE',
'Maximum model space distance between geometric entities at asserted c
onnectivities');
#99508=UNCERTAINTY_MEASURE_WITH_UNIT(LENGTH_MEASURE(0.01),#99527,
'DISTANCE_ACCURACY_VALUE',
'Maximum model space distance between geometric entities at asserted c
onnectivities');
#99512=(
GEOMETRIC_REPRESENTATION_CONTEXT(3)
GLOBAL_UNCERTAINTY_ASSIGNED_CONTEXT((#99494))
GLOBAL_UNIT_ASSIGNED_CONTEXT((#99527,#99529,#99530))
REPRESENTATION_CONTEXT('','3D')
);
#99526=(
GEOMETRIC_REPRESENTATION_CONTEXT(3)
GLOBAL_UNCERTAINTY_ASSIGNED_CONTEXT((#99508))
GLOBAL_UNIT_ASSIGNED_CONTEXT((#99527,#99529,#99530))
REPRESENTATION_CONTEXT('','3D')
);
#99527=(
LENGTH_UNIT()
NAMED_UNIT(*)
SI_UNIT(.MILLI.,.METRE.)
);
#99529=(
NAMED_UNIT(*)
PLANE_ANGLE_UNIT()
SI_UNIT($,.RADIAN.)
);
#99530=(
NAMED_UNIT(*)
SI_UNIT($,.STERADIAN.)
SOLID_ANGLE_UNIT()
);
#99534=SHAPE_DEFINITION_REPRESENTATION(#99551,#99627);
#99551=PRODUCT_DEFINITION_SHAPE('',$,#99645);
#99627=SHAPE_REPRESENTATION('',(#19430),#99512);
#99641=PRODUCT_DEFINITION_CONTEXT('part definition',#99694,'design');
#99645=PRODUCT_DEFINITION('Shaft','Shaft',#99662,#99641);
#99662=PRODUCT_DEFINITION_FORMATION('',$,#99699);
#99694=APPLICATION_CONTEXT(
'Core Data for Automotive Mechanical Design Process');
#99695=PRODUCT_CONTEXT('part definition',#99694,'mechanical');
#99699=PRODUCT('Shaft','Shaft','Shaft',(#99695));
#99716=PRESENTATION_STYLE_ASSIGNMENT((#99729));
#99729=SURFACE_STYLE_USAGE(.BOTH.,#99742);
#99742=SURFACE_SIDE_STYLE('',(#99755));
#99755=SURFACE_STYLE_FILL_AREA(#99768);
#99768=FILL_AREA_STYLE('Shaft gray',(#99781));
#99781=FILL_AREA_STYLE_COLOUR('Shaft gray',#99794);
#99794=COLOUR_RGB('Shaft gray',0.576470588235294,0.615686274509804,0.666666666666667);
ENDSEC;
END-ISO-10303-21;
